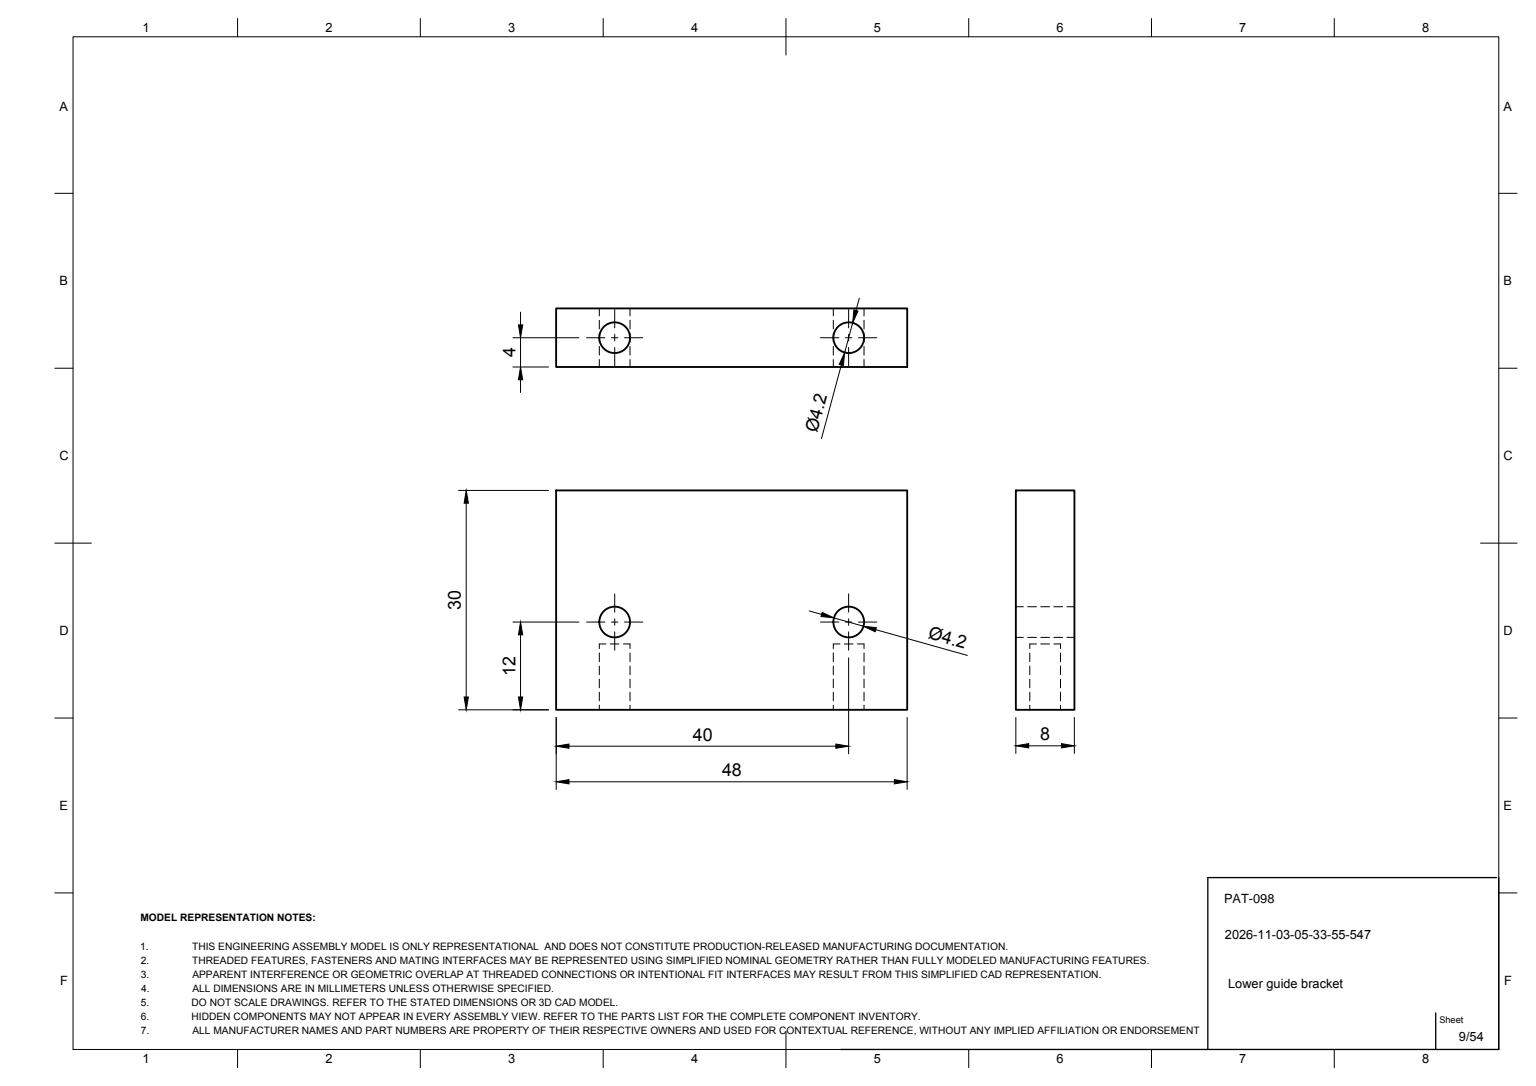
ISO-10303-21;
HEADER;
/* Generated by software containing ST-Developer
 * from STEP Tools, Inc. (www.steptools.com) 
 */

FILE_DESCRIPTION(
/* description */ ('Spring compression tester'),
/* implementation_level */ '2;1');

FILE_NAME(
/* name */ 'Lower guide bracket.step',
/* time_stamp */ '2026-10-28T03:24:11-07:00',
/* author */ (''),
/* organization */ (''),
/* preprocessor_version */ 'ST-DEVELOPER v20.2',
/* originating_system */ 'Autodesk Translation Framework v15.17.0.0',
/* authorisation */ '');

FILE_SCHEMA (('AUTOMOTIVE_DESIGN { 1 0 10303 214 3 1 1 }'));
ENDSEC;

DATA;
#10=MECHANICAL_DESIGN_GEOMETRIC_PRESENTATION_REPRESENTATION('',(#1110),#43521);
#990=SHAPE_REPRESENTATION_RELATIONSHIP('SRR','None',#43802,#1050);
#1050=ADVANCED_BREP_SHAPE_REPRESENTATION('',(#1185),#43462);
#1110=STYLED_ITEM('',(#44181),#1185);
#1185=MANIFOLD_SOLID_BREP('Body1',#18547);
#1321=FACE_BOUND('',#3396,.T.);
#1322=FACE_BOUND('',#3397,.T.);
#1323=FACE_BOUND('',#3400,.T.);
#1324=FACE_BOUND('',#3401,.T.);
#1325=FACE_BOUND('',#3405,.T.);
#1326=FACE_BOUND('',#3406,.T.);
#1645=PLANE('',#19478);
#1646=PLANE('',#19482);
#1647=PLANE('',#19489);
#1648=PLANE('',#19490);
#1649=PLANE('',#19491);
#1650=PLANE('',#19492);
#1651=PLANE('',#19493);
#1652=PLANE('',#19494);
#2268=FACE_OUTER_BOUND('',#3389,.T.);
#2269=FACE_OUTER_BOUND('',#3390,.T.);
#2270=FACE_OUTER_BOUND('',#3391,.T.);
#2271=FACE_OUTER_BOUND('',#3392,.T.);
#2272=FACE_OUTER_BOUND('',#3393,.T.);
#2273=FACE_OUTER_BOUND('',#3394,.T.);
#2274=FACE_OUTER_BOUND('',#3395,.T.);
#2275=FACE_OUTER_BOUND('',#3398,.T.);
#2276=FACE_OUTER_BOUND('',#3399,.T.);
#2277=FACE_OUTER_BOUND('',#3402,.T.);
#2278=FACE_OUTER_BOUND('',#3403,.T.);
#2279=FACE_OUTER_BOUND('',#3404,.T.);
#3389=EDGE_LOOP('',(#12661,#12662,#12663,#12664));
#3390=EDGE_LOOP('',(#12665));
#3391=EDGE_LOOP('',(#12666,#12667,#12668,#12669));
#3392=EDGE_LOOP('',(#12670));
#3393=EDGE_LOOP('',(#12671,#12672,#12673,#12674));
#3394=EDGE_LOOP('',(#12675,#12676,#12677,#12678));
#3395=EDGE_LOOP('',(#12679,#12680,#12681,#12682));
#3396=EDGE_LOOP('',(#12683));
#3397=EDGE_LOOP('',(#12684));
#3398=EDGE_LOOP('',(#12685,#12686,#12687,#12688));
#3399=EDGE_LOOP('',(#12689,#12690,#12691,#12692));
#3400=EDGE_LOOP('',(#12693));
#3401=EDGE_LOOP('',(#12694));
#3402=EDGE_LOOP('',(#12695,#12696,#12697,#12698));
#3403=EDGE_LOOP('',(#12699,#12700,#12701,#12702));
#3404=EDGE_LOOP('',(#12703,#12704,#12705,#12706));
#3405=EDGE_LOOP('',(#12707));
#3406=EDGE_LOOP('',(#12708));
#4744=LINE('',#26933,#6176);
#4745=LINE('',#26940,#6177);
#4746=LINE('',#26947,#6178);
#4747=LINE('',#26953,#6179);
#4748=LINE('',#26958,#6180);
#4749=LINE('',#26960,#6181);
#4750=LINE('',#26962,#6182);
#4751=LINE('',#26963,#6183);
#4752=LINE('',#26966,#6184);
#4753=LINE('',#26968,#6185);
#4754=LINE('',#26969,#6186);
#4755=LINE('',#26972,#6187);
#4756=LINE('',#26974,#6188);
#4757=LINE('',#26975,#6189);
#4758=LINE('',#26977,#6190);
#4759=LINE('',#26978,#6191);
#6176=VECTOR('',#21720,0.21);
#6177=VECTOR('',#21729,0.21);
#6178=VECTOR('',#21738,0.21);
#6179=VECTOR('',#21745,0.21);
#6180=VECTOR('',#21750,1.);
#6181=VECTOR('',#21751,1.);
#6182=VECTOR('',#21752,1.);
#6183=VECTOR('',#21753,1.);
#6184=VECTOR('',#21756,1.);
#6185=VECTOR('',#21757,1.);
#6186=VECTOR('',#21758,1.);
#6187=VECTOR('',#21761,1.);
#6188=VECTOR('',#21762,1.);
#6189=VECTOR('',#21763,1.);
#6190=VECTOR('',#21766,1.);
#6191=VECTOR('',#21767,1.);
#7554=CIRCLE('',#19476,0.21);
#7555=CIRCLE('',#19477,0.21);
#7556=CIRCLE('',#19480,0.21);
#7557=CIRCLE('',#19481,0.21);
#7558=CIRCLE('',#19484,0.21);
#7559=CIRCLE('',#19485,0.21);
#7560=CIRCLE('',#19487,0.21);
#7561=CIRCLE('',#19488,0.21);
#8284=VERTEX_POINT('',#26930);
#8285=VERTEX_POINT('',#26932);
#8286=VERTEX_POINT('',#26937);
#8287=VERTEX_POINT('',#26939);
#8288=VERTEX_POINT('',#26944);
#8289=VERTEX_POINT('',#26946);
#8290=VERTEX_POINT('',#26950);
#8291=VERTEX_POINT('',#26952);
#8292=VERTEX_POINT('',#26956);
#8293=VERTEX_POINT('',#26957);
#8294=VERTEX_POINT('',#26959);
#8295=VERTEX_POINT('',#26961);
#8296=VERTEX_POINT('',#26965);
#8297=VERTEX_POINT('',#26967);
#8298=VERTEX_POINT('',#26971);
#8299=VERTEX_POINT('',#26973);
#9995=EDGE_CURVE('',#8284,#8284,#7554,.T.);
#9996=EDGE_CURVE('',#8284,#8285,#4744,.T.);
#9997=EDGE_CURVE('',#8285,#8285,#7555,.T.);
#9998=EDGE_CURVE('',#8286,#8286,#7556,.T.);
#9999=EDGE_CURVE('',#8286,#8287,#4745,.T.);
#10000=EDGE_CURVE('',#8287,#8287,#7557,.T.);
#10001=EDGE_CURVE('',#8288,#8288,#7558,.T.);
#10002=EDGE_CURVE('',#8288,#8289,#4746,.T.);
#10003=EDGE_CURVE('',#8289,#8289,#7559,.T.);
#10004=EDGE_CURVE('',#8290,#8290,#7560,.T.);
#10005=EDGE_CURVE('',#8290,#8291,#4747,.T.);
#10006=EDGE_CURVE('',#8291,#8291,#7561,.T.);
#10007=EDGE_CURVE('',#8292,#8293,#4748,.T.);
#10008=EDGE_CURVE('',#8293,#8294,#4749,.T.);
#10009=EDGE_CURVE('',#8295,#8294,#4750,.T.);
#10010=EDGE_CURVE('',#8292,#8295,#4751,.T.);
#10011=EDGE_CURVE('',#8296,#8292,#4752,.T.);
#10012=EDGE_CURVE('',#8297,#8295,#4753,.T.);
#10013=EDGE_CURVE('',#8296,#8297,#4754,.T.);
#10014=EDGE_CURVE('',#8298,#8296,#4755,.T.);
#10015=EDGE_CURVE('',#8299,#8297,#4756,.T.);
#10016=EDGE_CURVE('',#8298,#8299,#4757,.T.);
#10017=EDGE_CURVE('',#8293,#8298,#4758,.T.);
#10018=EDGE_CURVE('',#8294,#8299,#4759,.T.);
#12661=ORIENTED_EDGE('',*,*,#9995,.F.);
#12662=ORIENTED_EDGE('',*,*,#9996,.T.);
#12663=ORIENTED_EDGE('',*,*,#9997,.T.);
#12664=ORIENTED_EDGE('',*,*,#9996,.F.);
#12665=ORIENTED_EDGE('',*,*,#9997,.F.);
#12666=ORIENTED_EDGE('',*,*,#9998,.F.);
#12667=ORIENTED_EDGE('',*,*,#9999,.T.);
#12668=ORIENTED_EDGE('',*,*,#10000,.T.);
#12669=ORIENTED_EDGE('',*,*,#9999,.F.);
#12670=ORIENTED_EDGE('',*,*,#10000,.F.);
#12671=ORIENTED_EDGE('',*,*,#10001,.F.);
#12672=ORIENTED_EDGE('',*,*,#10002,.T.);
#12673=ORIENTED_EDGE('',*,*,#10003,.F.);
#12674=ORIENTED_EDGE('',*,*,#10002,.F.);
#12675=ORIENTED_EDGE('',*,*,#10004,.F.);
#12676=ORIENTED_EDGE('',*,*,#10005,.T.);
#12677=ORIENTED_EDGE('',*,*,#10006,.F.);
#12678=ORIENTED_EDGE('',*,*,#10005,.F.);
#12679=ORIENTED_EDGE('',*,*,#10007,.T.);
#12680=ORIENTED_EDGE('',*,*,#10008,.T.);
#12681=ORIENTED_EDGE('',*,*,#10009,.F.);
#12682=ORIENTED_EDGE('',*,*,#10010,.F.);
#12683=ORIENTED_EDGE('',*,*,#10003,.T.);
#12684=ORIENTED_EDGE('',*,*,#10006,.T.);
#12685=ORIENTED_EDGE('',*,*,#10011,.T.);
#12686=ORIENTED_EDGE('',*,*,#10010,.T.);
#12687=ORIENTED_EDGE('',*,*,#10012,.F.);
#12688=ORIENTED_EDGE('',*,*,#10013,.F.);
#12689=ORIENTED_EDGE('',*,*,#10014,.T.);
#12690=ORIENTED_EDGE('',*,*,#10013,.T.);
#12691=ORIENTED_EDGE('',*,*,#10015,.F.);
#12692=ORIENTED_EDGE('',*,*,#10016,.F.);
#12693=ORIENTED_EDGE('',*,*,#10001,.T.);
#12694=ORIENTED_EDGE('',*,*,#10004,.T.);
#12695=ORIENTED_EDGE('',*,*,#10017,.T.);
#12696=ORIENTED_EDGE('',*,*,#10016,.T.);
#12697=ORIENTED_EDGE('',*,*,#10018,.F.);
#12698=ORIENTED_EDGE('',*,*,#10008,.F.);
#12699=ORIENTED_EDGE('',*,*,#10018,.T.);
#12700=ORIENTED_EDGE('',*,*,#10015,.T.);
#12701=ORIENTED_EDGE('',*,*,#10012,.T.);
#12702=ORIENTED_EDGE('',*,*,#10009,.T.);
#12703=ORIENTED_EDGE('',*,*,#10017,.F.);
#12704=ORIENTED_EDGE('',*,*,#10007,.F.);
#12705=ORIENTED_EDGE('',*,*,#10011,.F.);
#12706=ORIENTED_EDGE('',*,*,#10014,.F.);
#12707=ORIENTED_EDGE('',*,*,#9995,.T.);
#12708=ORIENTED_EDGE('',*,*,#9998,.T.);
#17147=CYLINDRICAL_SURFACE('',#19475,0.21);
#17148=CYLINDRICAL_SURFACE('',#19479,0.21);
#17149=CYLINDRICAL_SURFACE('',#19483,0.21);
#17150=CYLINDRICAL_SURFACE('',#19486,0.21);
#17592=ADVANCED_FACE('',(#2268),#17147,.F.);
#17593=ADVANCED_FACE('',(#2269),#1645,.F.);
#17594=ADVANCED_FACE('',(#2270),#17148,.F.);
#17595=ADVANCED_FACE('',(#2271),#1646,.F.);
#17596=ADVANCED_FACE('',(#2272),#17149,.F.);
#17597=ADVANCED_FACE('',(#2273),#17150,.F.);
#17598=ADVANCED_FACE('',(#2274,#1321,#1322),#1647,.T.);
#17599=ADVANCED_FACE('',(#2275),#1648,.T.);
#17600=ADVANCED_FACE('',(#2276,#1323,#1324),#1649,.T.);
#17601=ADVANCED_FACE('',(#2277),#1650,.T.);
#17602=ADVANCED_FACE('',(#2278),#1651,.T.);
#17603=ADVANCED_FACE('',(#2279,#1325,#1326),#1652,.F.);
#18547=CLOSED_SHELL('',(#17592,#17593,#17594,#17595,#17596,#17597,#17598,
#17599,#17600,#17601,#17602,#17603));
#19474=AXIS2_PLACEMENT_3D('',#26928,#21714,#21715);
#19475=AXIS2_PLACEMENT_3D('',#26929,#21716,#21717);
#19476=AXIS2_PLACEMENT_3D('',#26931,#21718,#21719);
#19477=AXIS2_PLACEMENT_3D('',#26934,#21721,#21722);
#19478=AXIS2_PLACEMENT_3D('',#26935,#21723,#21724);
#19479=AXIS2_PLACEMENT_3D('',#26936,#21725,#21726);
#19480=AXIS2_PLACEMENT_3D('',#26938,#21727,#21728);
#19481=AXIS2_PLACEMENT_3D('',#26941,#21730,#21731);
#19482=AXIS2_PLACEMENT_3D('',#26942,#21732,#21733);
#19483=AXIS2_PLACEMENT_3D('',#26943,#21734,#21735);
#19484=AXIS2_PLACEMENT_3D('',#26945,#21736,#21737);
#19485=AXIS2_PLACEMENT_3D('',#26948,#21739,#21740);
#19486=AXIS2_PLACEMENT_3D('',#26949,#21741,#21742);
#19487=AXIS2_PLACEMENT_3D('',#26951,#21743,#21744);
#19488=AXIS2_PLACEMENT_3D('',#26954,#21746,#21747);
#19489=AXIS2_PLACEMENT_3D('',#26955,#21748,#21749);
#19490=AXIS2_PLACEMENT_3D('',#26964,#21754,#21755);
#19491=AXIS2_PLACEMENT_3D('',#26970,#21759,#21760);
#19492=AXIS2_PLACEMENT_3D('',#26976,#21764,#21765);
#19493=AXIS2_PLACEMENT_3D('',#26979,#21768,#21769);
#19494=AXIS2_PLACEMENT_3D('',#26980,#21770,#21771);
#21714=DIRECTION('axis',(0.,0.,1.));
#21715=DIRECTION('refdir',(1.,0.,0.));
#21716=DIRECTION('center_axis',(0.,0.,1.));
#21717=DIRECTION('ref_axis',(1.,0.,0.));
#21718=DIRECTION('center_axis',(0.,0.,1.));
#21719=DIRECTION('ref_axis',(1.,0.,0.));
#21720=DIRECTION('',(0.,0.,1.));
#21721=DIRECTION('center_axis',(0.,0.,1.));
#21722=DIRECTION('ref_axis',(1.,0.,0.));
#21723=DIRECTION('center_axis',(0.,0.,1.));
#21724=DIRECTION('ref_axis',(1.,0.,0.));
#21725=DIRECTION('center_axis',(0.,0.,1.));
#21726=DIRECTION('ref_axis',(1.,0.,0.));
#21727=DIRECTION('center_axis',(0.,0.,1.));
#21728=DIRECTION('ref_axis',(1.,0.,0.));
#21729=DIRECTION('',(0.,0.,1.));
#21730=DIRECTION('center_axis',(0.,0.,1.));
#21731=DIRECTION('ref_axis',(1.,0.,0.));
#21732=DIRECTION('center_axis',(0.,0.,1.));
#21733=DIRECTION('ref_axis',(1.,0.,0.));
#21734=DIRECTION('center_axis',(0.,1.,0.));
#21735=DIRECTION('ref_axis',(1.,0.,0.));
#21736=DIRECTION('center_axis',(0.,1.,0.));
#21737=DIRECTION('ref_axis',(1.,0.,0.));
#21738=DIRECTION('',(0.,1.,0.));
#21739=DIRECTION('center_axis',(0.,-1.,0.));
#21740=DIRECTION('ref_axis',(1.,0.,0.));
#21741=DIRECTION('center_axis',(0.,1.,0.));
#21742=DIRECTION('ref_axis',(1.,0.,0.));
#21743=DIRECTION('center_axis',(0.,1.,0.));
#21744=DIRECTION('ref_axis',(1.,0.,0.));
#21745=DIRECTION('',(0.,1.,0.));
#21746=DIRECTION('center_axis',(0.,-1.,0.));
#21747=DIRECTION('ref_axis',(1.,0.,0.));
#21748=DIRECTION('center_axis',(0.,1.,0.));
#21749=DIRECTION('ref_axis',(-1.,0.,0.));
#21750=DIRECTION('',(-1.,0.,0.));
#21751=DIRECTION('',(0.,0.,1.));
#21752=DIRECTION('',(-1.,0.,0.));
#21753=DIRECTION('',(0.,0.,1.));
#21754=DIRECTION('center_axis',(1.,0.,0.));
#21755=DIRECTION('ref_axis',(0.,1.,0.));
#21756=DIRECTION('',(0.,1.,0.));
#21757=DIRECTION('',(0.,1.,0.));
#21758=DIRECTION('',(0.,0.,1.));
#21759=DIRECTION('center_axis',(0.,-1.,0.));
#21760=DIRECTION('ref_axis',(1.,0.,0.));
#21761=DIRECTION('',(1.,0.,0.));
#21762=DIRECTION('',(1.,0.,0.));
#21763=DIRECTION('',(0.,0.,1.));
#21764=DIRECTION('center_axis',(-1.,0.,0.));
#21765=DIRECTION('ref_axis',(0.,-1.,0.));
#21766=DIRECTION('',(0.,-1.,0.));
#21767=DIRECTION('',(0.,-1.,0.));
#21768=DIRECTION('center_axis',(0.,0.,1.));
#21769=DIRECTION('ref_axis',(1.,0.,0.));
#21770=DIRECTION('center_axis',(0.,0.,1.));
#21771=DIRECTION('ref_axis',(1.,0.,0.));
#26928=CARTESIAN_POINT('',(0.,0.,0.));
#26929=CARTESIAN_POINT('Origin',(-7.6,2.7,-0.1));
#26930=CARTESIAN_POINT('',(-7.81,2.7,0.));
#26931=CARTESIAN_POINT('Origin',(-7.6,2.7,0.));
#26932=CARTESIAN_POINT('',(-7.81,2.7,0.9));
#26933=CARTESIAN_POINT('',(-7.81,2.7,-0.1));
#26934=CARTESIAN_POINT('Origin',(-7.6,2.7,0.9));
#26935=CARTESIAN_POINT('Origin',(-7.6,2.7,0.9));
#26936=CARTESIAN_POINT('Origin',(-4.4,2.7,-0.1));
#26937=CARTESIAN_POINT('',(-4.61,2.7,0.));
#26938=CARTESIAN_POINT('Origin',(-4.4,2.7,0.));
#26939=CARTESIAN_POINT('',(-4.61,2.7,0.9));
#26940=CARTESIAN_POINT('',(-4.61,2.7,-0.1));
#26941=CARTESIAN_POINT('Origin',(-4.4,2.7,0.9));
#26942=CARTESIAN_POINT('Origin',(-4.4,2.7,0.9));
#26943=CARTESIAN_POINT('Origin',(-7.6,2.2,1.2));
#26944=CARTESIAN_POINT('',(-7.81,2.3,1.2));
#26945=CARTESIAN_POINT('Origin',(-7.6,2.3,1.2));
#26946=CARTESIAN_POINT('',(-7.81,3.1,1.2));
#26947=CARTESIAN_POINT('',(-7.81,2.2,1.2));
#26948=CARTESIAN_POINT('Origin',(-7.6,3.1,1.2));
#26949=CARTESIAN_POINT('Origin',(-4.4,2.2,1.2));
#26950=CARTESIAN_POINT('',(-4.61,2.3,1.2));
#26951=CARTESIAN_POINT('Origin',(-4.4,2.3,1.2));
#26952=CARTESIAN_POINT('',(-4.61,3.1,1.2));
#26953=CARTESIAN_POINT('',(-4.61,2.2,1.2));
#26954=CARTESIAN_POINT('Origin',(-4.4,3.1,1.2));
#26955=CARTESIAN_POINT('Origin',(-3.6,3.1,0.));
#26956=CARTESIAN_POINT('',(-3.6,3.1,0.));
#26957=CARTESIAN_POINT('',(-8.4,3.1,0.));
#26958=CARTESIAN_POINT('',(-3.6,3.1,0.));
#26959=CARTESIAN_POINT('',(-8.4,3.1,3.));
#26960=CARTESIAN_POINT('',(-8.4,3.1,0.));
#26961=CARTESIAN_POINT('',(-3.6,3.1,3.));
#26962=CARTESIAN_POINT('',(-3.6,3.1,3.));
#26963=CARTESIAN_POINT('',(-3.6,3.1,0.));
#26964=CARTESIAN_POINT('Origin',(-3.6,2.3,0.));
#26965=CARTESIAN_POINT('',(-3.6,2.3,0.));
#26966=CARTESIAN_POINT('',(-3.6,2.3,0.));
#26967=CARTESIAN_POINT('',(-3.6,2.3,3.));
#26968=CARTESIAN_POINT('',(-3.6,2.3,3.));
#26969=CARTESIAN_POINT('',(-3.6,2.3,0.));
#26970=CARTESIAN_POINT('Origin',(-8.4,2.3,0.));
#26971=CARTESIAN_POINT('',(-8.4,2.3,0.));
#26972=CARTESIAN_POINT('',(-8.4,2.3,0.));
#26973=CARTESIAN_POINT('',(-8.4,2.3,3.));
#26974=CARTESIAN_POINT('',(-8.4,2.3,3.));
#26975=CARTESIAN_POINT('',(-8.4,2.3,0.));
#26976=CARTESIAN_POINT('Origin',(-8.4,3.1,0.));
#26977=CARTESIAN_POINT('',(-8.4,3.1,0.));
#26978=CARTESIAN_POINT('',(-8.4,3.1,3.));
#26979=CARTESIAN_POINT('Origin',(-6.,2.7,3.));
#26980=CARTESIAN_POINT('Origin',(-6.,2.7,0.));
#43394=UNCERTAINTY_MEASURE_WITH_UNIT(LENGTH_MEASURE(0.001),#43522,
'DISTANCE_ACCURACY_VALUE',
'Maximum model space distance between geometric entities at asserted c
onnectivities');
#43453=UNCERTAINTY_MEASURE_WITH_UNIT(LENGTH_MEASURE(0.001),#43522,
'DISTANCE_ACCURACY_VALUE',
'Maximum model space distance between geometric entities at asserted c
onnectivities');
#43462=(
GEOMETRIC_REPRESENTATION_CONTEXT(3)
GLOBAL_UNCERTAINTY_ASSIGNED_CONTEXT((#43394))
GLOBAL_UNIT_ASSIGNED_CONTEXT((#43522,#43524,#43525))
REPRESENTATION_CONTEXT('','3D')
);
#43521=(
GEOMETRIC_REPRESENTATION_CONTEXT(3)
GLOBAL_UNCERTAINTY_ASSIGNED_CONTEXT((#43453))
GLOBAL_UNIT_ASSIGNED_CONTEXT((#43522,#43524,#43525))
REPRESENTATION_CONTEXT('','3D')
);
#43522=(
LENGTH_UNIT()
NAMED_UNIT(*)
SI_UNIT(.CENTI.,.METRE.)
);
#43524=(
NAMED_UNIT(*)
PLANE_ANGLE_UNIT()
SI_UNIT($,.RADIAN.)
);
#43525=(
NAMED_UNIT(*)
SI_UNIT($,.STERADIAN.)
SOLID_ANGLE_UNIT()
);
#43534=SHAPE_DEFINITION_REPRESENTATION(#43601,#43802);
#43601=PRODUCT_DEFINITION_SHAPE('',$,#43870);
#43802=SHAPE_REPRESENTATION('',(#19474),#43462);
#43861=PRODUCT_DEFINITION_CONTEXT('part definition',#44064,'design');
#43870=PRODUCT_DEFINITION('Lower guide bracket','Lower guide bracket',#43937,
#43861);
#43937=PRODUCT_DEFINITION_FORMATION('',$,#44074);
#44064=APPLICATION_CONTEXT(
'Core Data for Automotive Mechanical Design Process');
#44065=PRODUCT_CONTEXT('part definition',#44064,'mechanical');
#44074=PRODUCT('Lower guide bracket','Lower guide bracket',
'Lower guide bracket',(#44065));
#44175=COLOUR_RGB('Dark Blue',0.08,0.2,0.34);
#44176=FILL_AREA_STYLE_COLOUR('',#44175);
#44177=FILL_AREA_STYLE('',(#44176));
#44178=SURFACE_STYLE_FILL_AREA(#44177);
#44179=SURFACE_SIDE_STYLE('',(#44178));
#44180=SURFACE_STYLE_USAGE(.BOTH.,#44179);
#44181=PRESENTATION_STYLE_ASSIGNMENT((#44180));
ENDSEC;
END-ISO-10303-21;
